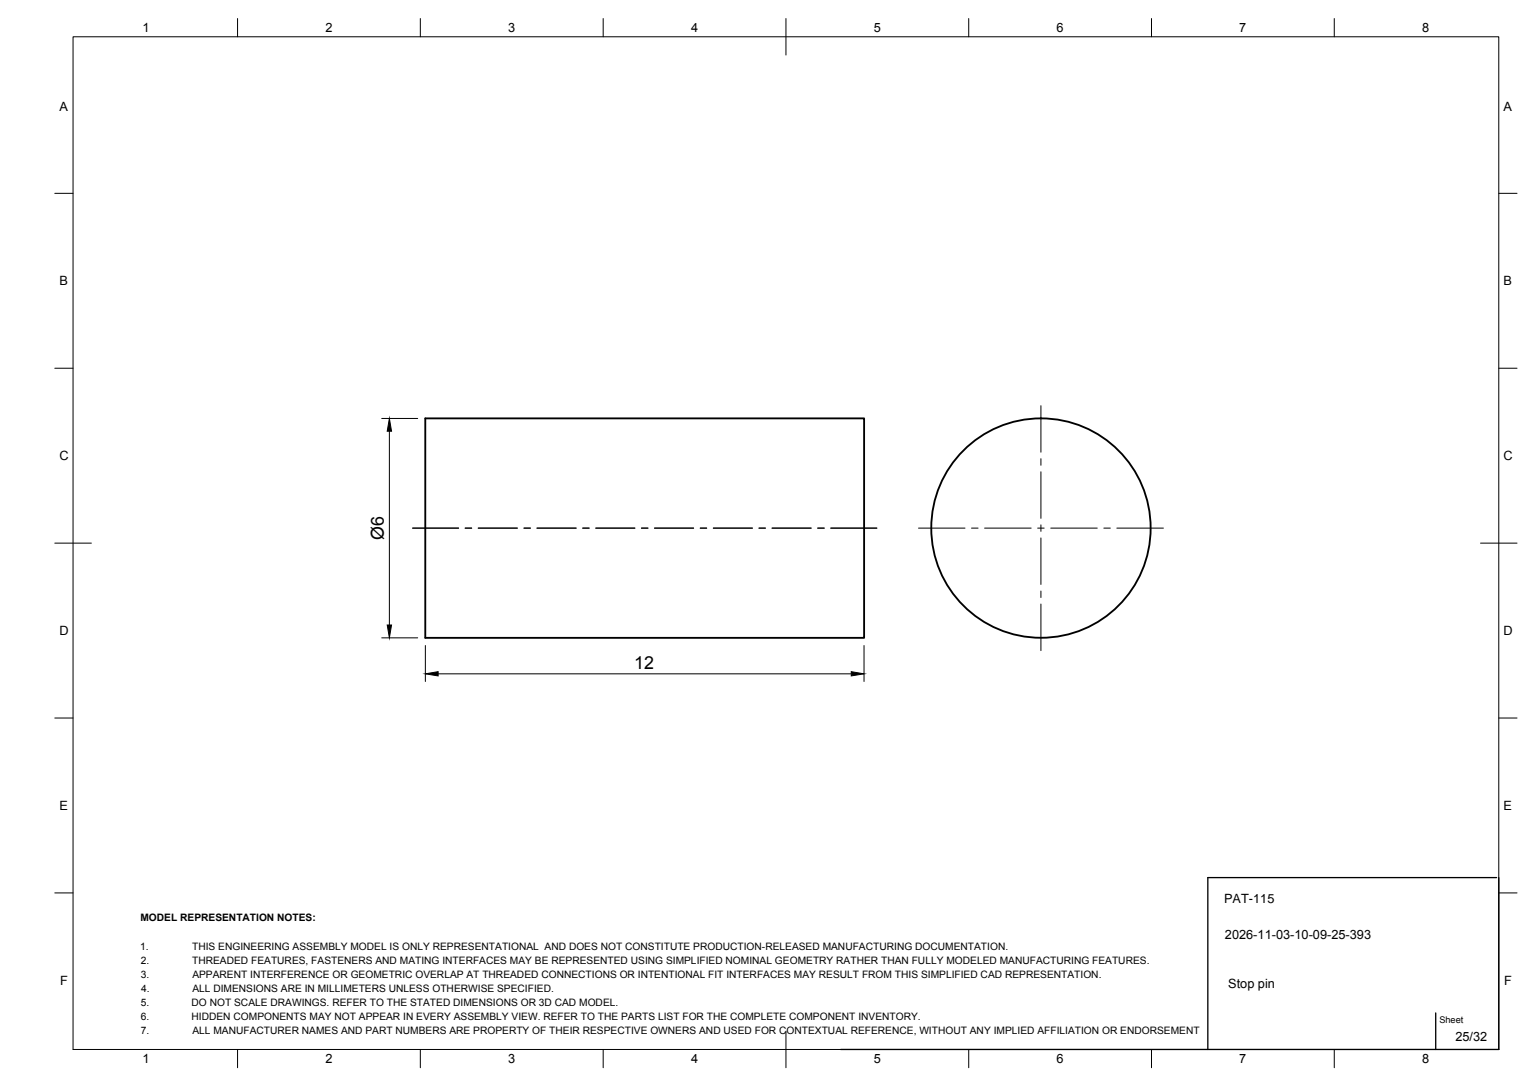
ISO-10303-21;
HEADER;
/* Generated by software containing ST-Developer
 * from STEP Tools, Inc. (www.steptools.com) 
 */

FILE_DESCRIPTION(
/* description */ ('Union bypass pipe loop'),
/* implementation_level */ '2;1');

FILE_NAME(
/* name */ 'Stop pin.step',
/* time_stamp */ '2026-10-27T21:00:29-07:00',
/* author */ (''),
/* organization */ (''),
/* preprocessor_version */ 'ST-DEVELOPER v20.2',
/* originating_system */ 'Autodesk Translation Framework v15.17.0.0',
/* authorisation */ '');

FILE_SCHEMA (('AUTOMOTIVE_DESIGN { 1 0 10303 214 3 1 1 }'));
ENDSEC;

DATA;
#10=MECHANICAL_DESIGN_GEOMETRIC_PRESENTATION_REPRESENTATION('',(#458),#10095);
#394=SHAPE_REPRESENTATION_RELATIONSHIP('SRR','None',#10263,#426);
#426=ADVANCED_BREP_SHAPE_REPRESENTATION('',(#488),#10075);
#458=STYLED_ITEM('',(#10500),#488);
#488=MANIFOLD_SOLID_BREP('Body1',#5531);
#719=PLANE('',#6186);
#720=PLANE('',#6187);
#981=FACE_OUTER_BOUND('',#1379,.T.);
#982=FACE_OUTER_BOUND('',#1380,.T.);
#983=FACE_OUTER_BOUND('',#1381,.T.);
#1379=EDGE_LOOP('',(#4334,#4335,#4336,#4337));
#1380=EDGE_LOOP('',(#4338));
#1381=EDGE_LOOP('',(#4339));
#1794=LINE('',#9108,#2170);
#2170=VECTOR('',#7350,0.3);
#2490=CIRCLE('',#6184,0.3);
#2491=CIRCLE('',#6185,0.3);
#2826=VERTEX_POINT('',#9105);
#2827=VERTEX_POINT('',#9107);
#3365=EDGE_CURVE('',#2826,#2826,#2490,.T.);
#3366=EDGE_CURVE('',#2826,#2827,#1794,.T.);
#3367=EDGE_CURVE('',#2827,#2827,#2491,.T.);
#4334=ORIENTED_EDGE('',*,*,#3365,.F.);
#4335=ORIENTED_EDGE('',*,*,#3366,.T.);
#4336=ORIENTED_EDGE('',*,*,#3367,.T.);
#4337=ORIENTED_EDGE('',*,*,#3366,.F.);
#4338=ORIENTED_EDGE('',*,*,#3365,.T.);
#4339=ORIENTED_EDGE('',*,*,#3367,.F.);
#5128=CYLINDRICAL_SURFACE('',#6183,0.3);
#5330=ADVANCED_FACE('',(#981),#5128,.T.);
#5331=ADVANCED_FACE('',(#982),#719,.T.);
#5332=ADVANCED_FACE('',(#983),#720,.F.);
#5531=CLOSED_SHELL('',(#5330,#5331,#5332));
#6182=AXIS2_PLACEMENT_3D('',#9103,#7344,#7345);
#6183=AXIS2_PLACEMENT_3D('',#9104,#7346,#7347);
#6184=AXIS2_PLACEMENT_3D('',#9106,#7348,#7349);
#6185=AXIS2_PLACEMENT_3D('',#9109,#7351,#7352);
#6186=AXIS2_PLACEMENT_3D('',#9110,#7353,#7354);
#6187=AXIS2_PLACEMENT_3D('',#9111,#7355,#7356);
#7344=DIRECTION('axis',(0.,0.,1.));
#7345=DIRECTION('refdir',(1.,0.,0.));
#7346=DIRECTION('center_axis',(0.,0.,1.));
#7347=DIRECTION('ref_axis',(1.,0.,0.));
#7348=DIRECTION('center_axis',(0.,0.,1.));
#7349=DIRECTION('ref_axis',(1.,0.,0.));
#7350=DIRECTION('',(0.,0.,-1.));
#7351=DIRECTION('center_axis',(0.,0.,1.));
#7352=DIRECTION('ref_axis',(1.,0.,0.));
#7353=DIRECTION('center_axis',(0.,0.,1.));
#7354=DIRECTION('ref_axis',(1.,0.,0.));
#7355=DIRECTION('center_axis',(0.,0.,1.));
#7356=DIRECTION('ref_axis',(1.,0.,0.));
#9103=CARTESIAN_POINT('',(0.,0.,0.));
#9104=CARTESIAN_POINT('Origin',(3.,1.1,8.2));
#9105=CARTESIAN_POINT('',(2.7,1.1,9.4));
#9106=CARTESIAN_POINT('Origin',(3.,1.1,9.4));
#9107=CARTESIAN_POINT('',(2.7,1.1,8.2));
#9108=CARTESIAN_POINT('',(2.7,1.1,8.2));
#9109=CARTESIAN_POINT('Origin',(3.,1.1,8.2));
#9110=CARTESIAN_POINT('Origin',(3.,1.1,9.4));
#9111=CARTESIAN_POINT('Origin',(3.,1.1,8.2));
#10038=UNCERTAINTY_MEASURE_WITH_UNIT(LENGTH_MEASURE(0.001),#10096,
'DISTANCE_ACCURACY_VALUE',
'Maximum model space distance between geometric entities at asserted c
onnectivities');
#10058=UNCERTAINTY_MEASURE_WITH_UNIT(LENGTH_MEASURE(0.001),#10096,
'DISTANCE_ACCURACY_VALUE',
'Maximum model space distance between geometric entities at asserted c
onnectivities');
#10075=(
GEOMETRIC_REPRESENTATION_CONTEXT(3)
GLOBAL_UNCERTAINTY_ASSIGNED_CONTEXT((#10038))
GLOBAL_UNIT_ASSIGNED_CONTEXT((#10096,#10098,#10099))
REPRESENTATION_CONTEXT('','3D')
);
#10095=(
GEOMETRIC_REPRESENTATION_CONTEXT(3)
GLOBAL_UNCERTAINTY_ASSIGNED_CONTEXT((#10058))
GLOBAL_UNIT_ASSIGNED_CONTEXT((#10096,#10098,#10099))
REPRESENTATION_CONTEXT('','3D')
);
#10096=(
LENGTH_UNIT()
NAMED_UNIT(*)
SI_UNIT(.CENTI.,.METRE.)
);
#10098=(
NAMED_UNIT(*)
PLANE_ANGLE_UNIT()
SI_UNIT($,.RADIAN.)
);
#10099=(
NAMED_UNIT(*)
SI_UNIT($,.STERADIAN.)
SOLID_ANGLE_UNIT()
);
#10116=SHAPE_DEFINITION_REPRESENTATION(#10152,#10263);
#10152=PRODUCT_DEFINITION_SHAPE('',$,#10300);
#10263=SHAPE_REPRESENTATION('',(#6182),#10075);
#10283=PRODUCT_DEFINITION_CONTEXT('part definition',#10393,'design');
#10300=PRODUCT_DEFINITION('Stop pin','Stop pin',#10336,#10283);
#10336=PRODUCT_DEFINITION_FORMATION('',$,#10411);
#10393=APPLICATION_CONTEXT(
'Core Data for Automotive Mechanical Design Process');
#10394=PRODUCT_CONTEXT('part definition',#10393,'mechanical');
#10411=PRODUCT('Stop pin','Stop pin','Stop pin',(#10394));
#10494=COLOUR_RGB('Grey',0.48,0.52,0.57);
#10495=FILL_AREA_STYLE_COLOUR('',#10494);
#10496=FILL_AREA_STYLE('',(#10495));
#10497=SURFACE_STYLE_FILL_AREA(#10496);
#10498=SURFACE_SIDE_STYLE('',(#10497));
#10499=SURFACE_STYLE_USAGE(.BOTH.,#10498);
#10500=PRESENTATION_STYLE_ASSIGNMENT((#10499));
ENDSEC;
END-ISO-10303-21;
